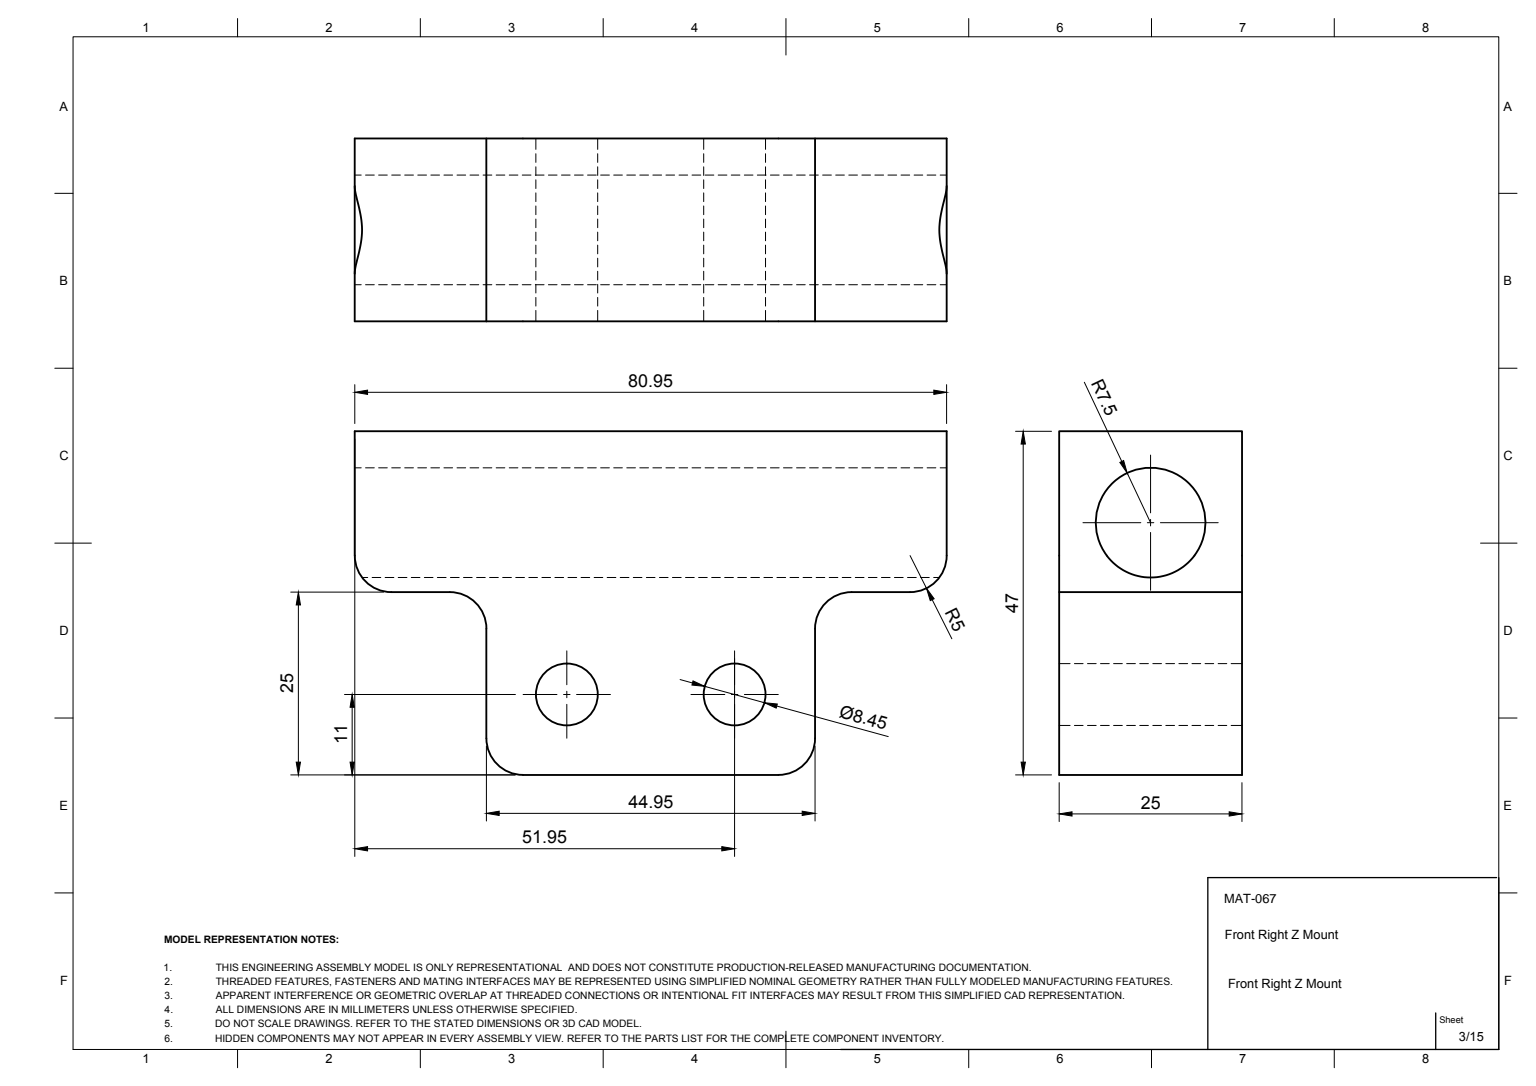
ISO-10303-21;
HEADER;
/* Generated by software containing ST-Developer
 * from STEP Tools, Inc. (www.steptools.com) 
 */

FILE_DESCRIPTION(
/* description */ ('CAx-IF Rec.Pracs.---Representation and Presentation of Product Manufa
cturing Information (PMI)---4.0---2014-10-13'),
/* implementation_level */ '2;1');

FILE_NAME(
/* name */ 'Front Right Z Mount.step',
/* time_stamp */ '2026-10-24T16:02:03-07:00',
/* author */ (''),
/* organization */ (''),
/* preprocessor_version */ 'ST-DEVELOPER v20.2',
/* originating_system */ 'Autodesk Translation Framework v15.17.0.0',
/* authorisation */ '');

FILE_SCHEMA (('AP242_MANAGED_MODEL_BASED_3D_ENGINEERING_MIM_LF { 1 0 10303 442 2 1 4 }'));
ENDSEC;

DATA;
#10=MECHANICAL_DESIGN_GEOMETRIC_PRESENTATION_REPRESENTATION('',(#349),#6348);
#327=SHAPE_REPRESENTATION_RELATIONSHIP('SRR','None',#6477,#338);
#338=ADVANCED_BREP_SHAPE_REPRESENTATION('',(#360),#6325);
#349=STYLED_ITEM('',(#6601),#360);
#360=MANIFOLD_SOLID_BREP('Body1',#3388);
#371=B_SPLINE_CURVE_WITH_KNOTS('',3,(#5227,#5228,#5229,#5230,#5231,#5232,
#5233,#5234,#5235,#5236,#5237,#5238,#5239,#5240,#5241,#5242,#5243,#5244),
 .UNSPECIFIED.,.F.,.F.,(4,2,2,2,2,2,2,2,4),(3.70111917994048,3.77979672158967,
4.08163951097076,4.2325609056613,4.38348230035184,4.53440369504239,4.68532508973293,
4.98716787911402,5.06584542076321),.UNSPECIFIED.);
#372=B_SPLINE_CURVE_WITH_KNOTS('',3,(#5245,#5246,#5247,#5248,#5249,#5250,
#5251,#5252,#5253,#5254,#5255,#5256,#5257,#5258,#5259,#5260,#5261,#5262),
 .UNSPECIFIED.,.F.,.F.,(4,2,2,2,2,2,2,2,4),(0.778797646372586,0.857475188021775,
1.15931797740286,1.31023937209341,1.46116076678395,1.61208216147449,1.76300355616504,
2.06484634554612,2.14352388719531),.UNSPECIFIED.);
#385=CYLINDRICAL_SURFACE('',#3548,0.004225);
#386=CYLINDRICAL_SURFACE('',#3549,0.004225);
#387=CYLINDRICAL_SURFACE('',#3551,0.0075);
#388=CYLINDRICAL_SURFACE('',#3556,0.005);
#389=CYLINDRICAL_SURFACE('',#3557,0.005);
#390=CYLINDRICAL_SURFACE('',#3558,0.005);
#391=CYLINDRICAL_SURFACE('',#3559,0.005);
#392=CYLINDRICAL_SURFACE('',#3560,0.005);
#393=CYLINDRICAL_SURFACE('',#3561,0.005);
#464=FACE_BOUND('',#869,.T.);
#465=FACE_BOUND('',#870,.T.);
#466=FACE_BOUND('',#872,.T.);
#467=FACE_BOUND('',#873,.T.);
#506=CIRCLE('',#3525,0.0075);
#507=CIRCLE('',#3526,0.0075);
#508=CIRCLE('',#3528,0.0075);
#509=CIRCLE('',#3529,0.0075);
#510=CIRCLE('',#3531,0.005);
#511=CIRCLE('',#3532,0.005);
#512=CIRCLE('',#3533,0.005);
#513=CIRCLE('',#3534,0.005);
#514=CIRCLE('',#3535,0.005);
#515=CIRCLE('',#3536,0.005);
#516=CIRCLE('',#3537,0.004225);
#517=CIRCLE('',#3538,0.004225);
#518=CIRCLE('',#3540,0.005);
#519=CIRCLE('',#3541,0.005);
#520=CIRCLE('',#3542,0.005);
#521=CIRCLE('',#3543,0.005);
#522=CIRCLE('',#3544,0.005);
#523=CIRCLE('',#3545,0.005);
#524=CIRCLE('',#3546,0.004225);
#525=CIRCLE('',#3547,0.004225);
#694=FACE_OUTER_BOUND('',#865,.T.);
#695=FACE_OUTER_BOUND('',#866,.T.);
#696=FACE_OUTER_BOUND('',#867,.T.);
#697=FACE_OUTER_BOUND('',#868,.T.);
#698=FACE_OUTER_BOUND('',#871,.T.);
#699=FACE_OUTER_BOUND('',#874,.T.);
#700=FACE_OUTER_BOUND('',#875,.T.);
#701=FACE_OUTER_BOUND('',#876,.T.);
#702=FACE_OUTER_BOUND('',#877,.T.);
#703=FACE_OUTER_BOUND('',#878,.T.);
#704=FACE_OUTER_BOUND('',#879,.T.);
#705=FACE_OUTER_BOUND('',#880,.T.);
#706=FACE_OUTER_BOUND('',#881,.T.);
#707=FACE_OUTER_BOUND('',#882,.T.);
#708=FACE_OUTER_BOUND('',#883,.T.);
#709=FACE_OUTER_BOUND('',#884,.T.);
#710=FACE_OUTER_BOUND('',#885,.T.);
#711=FACE_OUTER_BOUND('',#886,.T.);
#712=FACE_OUTER_BOUND('',#887,.T.);
#865=EDGE_LOOP('',(#2267,#2268,#2269,#2270));
#866=EDGE_LOOP('',(#2271,#2272,#2273,#2274,#2275,#2276,#2277));
#867=EDGE_LOOP('',(#2278,#2279,#2280,#2281,#2282,#2283,#2284));
#868=EDGE_LOOP('',(#2285,#2286,#2287,#2288,#2289,#2290,#2291,#2292,#2293,
#2294,#2295,#2296,#2297,#2298));
#869=EDGE_LOOP('',(#2299));
#870=EDGE_LOOP('',(#2300));
#871=EDGE_LOOP('',(#2301,#2302,#2303,#2304,#2305,#2306,#2307,#2308,#2309,
#2310,#2311,#2312,#2313,#2314));
#872=EDGE_LOOP('',(#2315));
#873=EDGE_LOOP('',(#2316));
#874=EDGE_LOOP('',(#2317,#2318,#2319,#2320));
#875=EDGE_LOOP('',(#2321,#2322,#2323,#2324));
#876=EDGE_LOOP('',(#2325,#2326,#2327,#2328));
#877=EDGE_LOOP('',(#2329,#2330,#2331,#2332,#2333,#2334,#2335,#2336));
#878=EDGE_LOOP('',(#2337,#2338,#2339,#2340));
#879=EDGE_LOOP('',(#2341,#2342,#2343,#2344));
#880=EDGE_LOOP('',(#2345,#2346,#2347,#2348));
#881=EDGE_LOOP('',(#2349,#2350,#2351,#2352));
#882=EDGE_LOOP('',(#2353,#2354,#2355,#2356));
#883=EDGE_LOOP('',(#2357,#2358,#2359,#2360,#2361,#2362));
#884=EDGE_LOOP('',(#2363,#2364,#2365,#2366));
#885=EDGE_LOOP('',(#2367,#2368,#2369,#2370,#2371,#2372));
#886=EDGE_LOOP('',(#2373,#2374,#2375,#2376));
#887=EDGE_LOOP('',(#2377,#2378,#2379,#2380));
#1078=LINE('',#5136,#1311);
#1079=LINE('',#5138,#1312);
#1080=LINE('',#5140,#1313);
#1081=LINE('',#5141,#1314);
#1082=LINE('',#5145,#1315);
#1083=LINE('',#5147,#1316);
#1084=LINE('',#5149,#1317);
#1085=LINE('',#5151,#1318);
#1086=LINE('',#5156,#1319);
#1087=LINE('',#5160,#1320);
#1088=LINE('',#5162,#1321);
#1089=LINE('',#5164,#1322);
#1090=LINE('',#5166,#1323);
#1091=LINE('',#5171,#1324);
#1092=LINE('',#5176,#1325);
#1093=LINE('',#5180,#1326);
#1094=LINE('',#5182,#1327);
#1095=LINE('',#5186,#1328);
#1096=LINE('',#5190,#1329);
#1097=LINE('',#5199,#1330);
#1098=LINE('',#5203,#1331);
#1099=LINE('',#5205,#1332);
#1100=LINE('',#5209,#1333);
#1101=LINE('',#5213,#1334);
#1102=LINE('',#5221,#1335);
#1103=LINE('',#5223,#1336);
#1104=LINE('',#5226,#1337);
#1105=LINE('',#5264,#1338);
#1106=LINE('',#5265,#1339);
#1107=LINE('',#5267,#1340);
#1108=LINE('',#5268,#1341);
#1109=LINE('',#5270,#1342);
#1110=LINE('',#5271,#1343);
#1111=LINE('',#5273,#1344);
#1112=LINE('',#5274,#1345);
#1311=VECTOR('',#3986,1.);
#1312=VECTOR('',#3987,1.);
#1313=VECTOR('',#3988,1.);
#1314=VECTOR('',#3989,1.);
#1315=VECTOR('',#3992,1.);
#1316=VECTOR('',#3993,1.);
#1317=VECTOR('',#3994,1.);
#1318=VECTOR('',#3995,1.);
#1319=VECTOR('',#4000,1.);
#1320=VECTOR('',#4003,1.);
#1321=VECTOR('',#4004,1.);
#1322=VECTOR('',#4005,1.);
#1323=VECTOR('',#4006,1.);
#1324=VECTOR('',#4011,1.);
#1325=VECTOR('',#4016,1.);
#1326=VECTOR('',#4019,1.);
#1327=VECTOR('',#4022,1.);
#1328=VECTOR('',#4025,1.);
#1329=VECTOR('',#4028,1.);
#1330=VECTOR('',#4037,1.);
#1331=VECTOR('',#4040,1.);
#1332=VECTOR('',#4043,1.);
#1333=VECTOR('',#4046,1.);
#1334=VECTOR('',#4049,1.);
#1335=VECTOR('',#4060,0.004225);
#1336=VECTOR('',#4063,0.004225);
#1337=VECTOR('',#4068,0.0075);
#1338=VECTOR('',#4071,1.);
#1339=VECTOR('',#4072,1.);
#1340=VECTOR('',#4075,1.);
#1341=VECTOR('',#4076,1.);
#1342=VECTOR('',#4079,1.);
#1343=VECTOR('',#4080,1.);
#1344=VECTOR('',#4083,1.);
#1345=VECTOR('',#4084,1.);
#1544=VERTEX_POINT('',#5134);
#1545=VERTEX_POINT('',#5135);
#1546=VERTEX_POINT('',#5137);
#1547=VERTEX_POINT('',#5139);
#1548=VERTEX_POINT('',#5143);
#1549=VERTEX_POINT('',#5144);
#1550=VERTEX_POINT('',#5146);
#1551=VERTEX_POINT('',#5148);
#1552=VERTEX_POINT('',#5150);
#1553=VERTEX_POINT('',#5152);
#1554=VERTEX_POINT('',#5154);
#1555=VERTEX_POINT('',#5158);
#1556=VERTEX_POINT('',#5159);
#1557=VERTEX_POINT('',#5161);
#1558=VERTEX_POINT('',#5163);
#1559=VERTEX_POINT('',#5165);
#1560=VERTEX_POINT('',#5167);
#1561=VERTEX_POINT('',#5169);
#1562=VERTEX_POINT('',#5173);
#1563=VERTEX_POINT('',#5175);
#1564=VERTEX_POINT('',#5177);
#1565=VERTEX_POINT('',#5179);
#1566=VERTEX_POINT('',#5183);
#1567=VERTEX_POINT('',#5185);
#1568=VERTEX_POINT('',#5187);
#1569=VERTEX_POINT('',#5189);
#1570=VERTEX_POINT('',#5192);
#1571=VERTEX_POINT('',#5194);
#1572=VERTEX_POINT('',#5197);
#1573=VERTEX_POINT('',#5198);
#1574=VERTEX_POINT('',#5200);
#1575=VERTEX_POINT('',#5202);
#1576=VERTEX_POINT('',#5206);
#1577=VERTEX_POINT('',#5208);
#1578=VERTEX_POINT('',#5210);
#1579=VERTEX_POINT('',#5212);
#1580=VERTEX_POINT('',#5216);
#1581=VERTEX_POINT('',#5218);
#1832=EDGE_CURVE('',#1544,#1545,#1078,.T.);
#1833=EDGE_CURVE('',#1546,#1544,#1079,.F.);
#1834=EDGE_CURVE('',#1546,#1547,#1080,.T.);
#1835=EDGE_CURVE('',#1545,#1547,#1081,.T.);
#1836=EDGE_CURVE('',#1548,#1549,#1082,.T.);
#1837=EDGE_CURVE('',#1549,#1550,#1083,.T.);
#1838=EDGE_CURVE('',#1551,#1550,#1084,.T.);
#1839=EDGE_CURVE('',#1552,#1551,#1085,.F.);
#1840=EDGE_CURVE('',#1553,#1552,#506,.T.);
#1841=EDGE_CURVE('',#1554,#1553,#507,.T.);
#1842=EDGE_CURVE('',#1548,#1554,#1086,.F.);
#1843=EDGE_CURVE('',#1555,#1556,#1087,.T.);
#1844=EDGE_CURVE('',#1557,#1556,#1088,.T.);
#1845=EDGE_CURVE('',#1558,#1557,#1089,.T.);
#1846=EDGE_CURVE('',#1559,#1558,#1090,.T.);
#1847=EDGE_CURVE('',#1559,#1560,#508,.T.);
#1848=EDGE_CURVE('',#1560,#1561,#509,.T.);
#1849=EDGE_CURVE('',#1555,#1561,#1091,.T.);
#1850=EDGE_CURVE('',#1562,#1546,#510,.T.);
#1851=EDGE_CURVE('',#1562,#1563,#1092,.T.);
#1852=EDGE_CURVE('',#1564,#1563,#511,.F.);
#1853=EDGE_CURVE('',#1565,#1564,#1093,.T.);
#1854=EDGE_CURVE('',#1558,#1565,#512,.T.);
#1855=EDGE_CURVE('',#1557,#1549,#1094,.T.);
#1856=EDGE_CURVE('',#1566,#1548,#513,.T.);
#1857=EDGE_CURVE('',#1566,#1567,#1095,.T.);
#1858=EDGE_CURVE('',#1568,#1567,#514,.F.);
#1859=EDGE_CURVE('',#1569,#1568,#1096,.T.);
#1860=EDGE_CURVE('',#1547,#1569,#515,.T.);
#1861=EDGE_CURVE('',#1570,#1570,#516,.T.);
#1862=EDGE_CURVE('',#1571,#1571,#517,.T.);
#1863=EDGE_CURVE('',#1572,#1573,#1097,.T.);
#1864=EDGE_CURVE('',#1574,#1573,#518,.T.);
#1865=EDGE_CURVE('',#1575,#1574,#1098,.T.);
#1866=EDGE_CURVE('',#1551,#1575,#519,.F.);
#1867=EDGE_CURVE('',#1556,#1550,#1099,.T.);
#1868=EDGE_CURVE('',#1576,#1555,#520,.F.);
#1869=EDGE_CURVE('',#1576,#1577,#1100,.T.);
#1870=EDGE_CURVE('',#1578,#1577,#521,.T.);
#1871=EDGE_CURVE('',#1579,#1578,#1101,.T.);
#1872=EDGE_CURVE('',#1544,#1579,#522,.F.);
#1873=EDGE_CURVE('',#1572,#1545,#523,.F.);
#1874=EDGE_CURVE('',#1580,#1580,#524,.T.);
#1875=EDGE_CURVE('',#1581,#1581,#525,.T.);
#1876=EDGE_CURVE('',#1570,#1580,#1102,.T.);
#1877=EDGE_CURVE('',#1571,#1581,#1103,.T.);
#1878=EDGE_CURVE('',#1553,#1560,#1104,.T.);
#1879=EDGE_CURVE('',#1561,#1559,#371,.T.);
#1880=EDGE_CURVE('',#1554,#1552,#372,.T.);
#1881=EDGE_CURVE('',#1573,#1568,#1105,.T.);
#1882=EDGE_CURVE('',#1569,#1572,#1106,.F.);
#1883=EDGE_CURVE('',#1567,#1574,#1107,.F.);
#1884=EDGE_CURVE('',#1575,#1566,#1108,.T.);
#1885=EDGE_CURVE('',#1579,#1562,#1109,.T.);
#1886=EDGE_CURVE('',#1563,#1578,#1110,.F.);
#1887=EDGE_CURVE('',#1577,#1564,#1111,.T.);
#1888=EDGE_CURVE('',#1565,#1576,#1112,.F.);
#2267=ORIENTED_EDGE('',*,*,#1832,.F.);
#2268=ORIENTED_EDGE('',*,*,#1833,.F.);
#2269=ORIENTED_EDGE('',*,*,#1834,.T.);
#2270=ORIENTED_EDGE('',*,*,#1835,.F.);
#2271=ORIENTED_EDGE('',*,*,#1836,.T.);
#2272=ORIENTED_EDGE('',*,*,#1837,.T.);
#2273=ORIENTED_EDGE('',*,*,#1838,.F.);
#2274=ORIENTED_EDGE('',*,*,#1839,.F.);
#2275=ORIENTED_EDGE('',*,*,#1840,.F.);
#2276=ORIENTED_EDGE('',*,*,#1841,.F.);
#2277=ORIENTED_EDGE('',*,*,#1842,.F.);
#2278=ORIENTED_EDGE('',*,*,#1843,.T.);
#2279=ORIENTED_EDGE('',*,*,#1844,.F.);
#2280=ORIENTED_EDGE('',*,*,#1845,.F.);
#2281=ORIENTED_EDGE('',*,*,#1846,.F.);
#2282=ORIENTED_EDGE('',*,*,#1847,.T.);
#2283=ORIENTED_EDGE('',*,*,#1848,.T.);
#2284=ORIENTED_EDGE('',*,*,#1849,.F.);
#2285=ORIENTED_EDGE('',*,*,#1834,.F.);
#2286=ORIENTED_EDGE('',*,*,#1850,.F.);
#2287=ORIENTED_EDGE('',*,*,#1851,.T.);
#2288=ORIENTED_EDGE('',*,*,#1852,.F.);
#2289=ORIENTED_EDGE('',*,*,#1853,.F.);
#2290=ORIENTED_EDGE('',*,*,#1854,.F.);
#2291=ORIENTED_EDGE('',*,*,#1845,.T.);
#2292=ORIENTED_EDGE('',*,*,#1855,.T.);
#2293=ORIENTED_EDGE('',*,*,#1836,.F.);
#2294=ORIENTED_EDGE('',*,*,#1856,.F.);
#2295=ORIENTED_EDGE('',*,*,#1857,.T.);
#2296=ORIENTED_EDGE('',*,*,#1858,.F.);
#2297=ORIENTED_EDGE('',*,*,#1859,.F.);
#2298=ORIENTED_EDGE('',*,*,#1860,.F.);
#2299=ORIENTED_EDGE('',*,*,#1861,.T.);
#2300=ORIENTED_EDGE('',*,*,#1862,.T.);
#2301=ORIENTED_EDGE('',*,*,#1863,.T.);
#2302=ORIENTED_EDGE('',*,*,#1864,.F.);
#2303=ORIENTED_EDGE('',*,*,#1865,.F.);
#2304=ORIENTED_EDGE('',*,*,#1866,.F.);
#2305=ORIENTED_EDGE('',*,*,#1838,.T.);
#2306=ORIENTED_EDGE('',*,*,#1867,.F.);
#2307=ORIENTED_EDGE('',*,*,#1843,.F.);
#2308=ORIENTED_EDGE('',*,*,#1868,.F.);
#2309=ORIENTED_EDGE('',*,*,#1869,.T.);
#2310=ORIENTED_EDGE('',*,*,#1870,.F.);
#2311=ORIENTED_EDGE('',*,*,#1871,.F.);
#2312=ORIENTED_EDGE('',*,*,#1872,.F.);
#2313=ORIENTED_EDGE('',*,*,#1832,.T.);
#2314=ORIENTED_EDGE('',*,*,#1873,.F.);
#2315=ORIENTED_EDGE('',*,*,#1874,.F.);
#2316=ORIENTED_EDGE('',*,*,#1875,.F.);
#2317=ORIENTED_EDGE('',*,*,#1861,.F.);
#2318=ORIENTED_EDGE('',*,*,#1876,.T.);
#2319=ORIENTED_EDGE('',*,*,#1874,.T.);
#2320=ORIENTED_EDGE('',*,*,#1876,.F.);
#2321=ORIENTED_EDGE('',*,*,#1862,.F.);
#2322=ORIENTED_EDGE('',*,*,#1877,.T.);
#2323=ORIENTED_EDGE('',*,*,#1875,.T.);
#2324=ORIENTED_EDGE('',*,*,#1877,.F.);
#2325=ORIENTED_EDGE('',*,*,#1867,.T.);
#2326=ORIENTED_EDGE('',*,*,#1837,.F.);
#2327=ORIENTED_EDGE('',*,*,#1855,.F.);
#2328=ORIENTED_EDGE('',*,*,#1844,.T.);
#2329=ORIENTED_EDGE('',*,*,#1841,.T.);
#2330=ORIENTED_EDGE('',*,*,#1878,.T.);
#2331=ORIENTED_EDGE('',*,*,#1847,.F.);
#2332=ORIENTED_EDGE('',*,*,#1879,.F.);
#2333=ORIENTED_EDGE('',*,*,#1848,.F.);
#2334=ORIENTED_EDGE('',*,*,#1878,.F.);
#2335=ORIENTED_EDGE('',*,*,#1840,.T.);
#2336=ORIENTED_EDGE('',*,*,#1880,.F.);
#2337=ORIENTED_EDGE('',*,*,#1859,.T.);
#2338=ORIENTED_EDGE('',*,*,#1881,.F.);
#2339=ORIENTED_EDGE('',*,*,#1863,.F.);
#2340=ORIENTED_EDGE('',*,*,#1882,.F.);
#2341=ORIENTED_EDGE('',*,*,#1865,.T.);
#2342=ORIENTED_EDGE('',*,*,#1883,.F.);
#2343=ORIENTED_EDGE('',*,*,#1857,.F.);
#2344=ORIENTED_EDGE('',*,*,#1884,.F.);
#2345=ORIENTED_EDGE('',*,*,#1851,.F.);
#2346=ORIENTED_EDGE('',*,*,#1885,.F.);
#2347=ORIENTED_EDGE('',*,*,#1871,.T.);
#2348=ORIENTED_EDGE('',*,*,#1886,.F.);
#2349=ORIENTED_EDGE('',*,*,#1853,.T.);
#2350=ORIENTED_EDGE('',*,*,#1887,.F.);
#2351=ORIENTED_EDGE('',*,*,#1869,.F.);
#2352=ORIENTED_EDGE('',*,*,#1888,.F.);
#2353=ORIENTED_EDGE('',*,*,#1873,.T.);
#2354=ORIENTED_EDGE('',*,*,#1835,.T.);
#2355=ORIENTED_EDGE('',*,*,#1860,.T.);
#2356=ORIENTED_EDGE('',*,*,#1882,.T.);
#2357=ORIENTED_EDGE('',*,*,#1880,.T.);
#2358=ORIENTED_EDGE('',*,*,#1839,.T.);
#2359=ORIENTED_EDGE('',*,*,#1866,.T.);
#2360=ORIENTED_EDGE('',*,*,#1884,.T.);
#2361=ORIENTED_EDGE('',*,*,#1856,.T.);
#2362=ORIENTED_EDGE('',*,*,#1842,.T.);
#2363=ORIENTED_EDGE('',*,*,#1864,.T.);
#2364=ORIENTED_EDGE('',*,*,#1881,.T.);
#2365=ORIENTED_EDGE('',*,*,#1858,.T.);
#2366=ORIENTED_EDGE('',*,*,#1883,.T.);
#2367=ORIENTED_EDGE('',*,*,#1868,.T.);
#2368=ORIENTED_EDGE('',*,*,#1849,.T.);
#2369=ORIENTED_EDGE('',*,*,#1879,.T.);
#2370=ORIENTED_EDGE('',*,*,#1846,.T.);
#2371=ORIENTED_EDGE('',*,*,#1854,.T.);
#2372=ORIENTED_EDGE('',*,*,#1888,.T.);
#2373=ORIENTED_EDGE('',*,*,#1870,.T.);
#2374=ORIENTED_EDGE('',*,*,#1887,.T.);
#2375=ORIENTED_EDGE('',*,*,#1852,.T.);
#2376=ORIENTED_EDGE('',*,*,#1886,.T.);
#2377=ORIENTED_EDGE('',*,*,#1872,.T.);
#2378=ORIENTED_EDGE('',*,*,#1885,.T.);
#2379=ORIENTED_EDGE('',*,*,#1850,.T.);
#2380=ORIENTED_EDGE('',*,*,#1833,.T.);
#3137=PLANE('',#3523);
#3138=PLANE('',#3524);
#3139=PLANE('',#3527);
#3140=PLANE('',#3530);
#3141=PLANE('',#3539);
#3142=PLANE('',#3550);
#3143=PLANE('',#3552);
#3144=PLANE('',#3553);
#3145=PLANE('',#3554);
#3146=PLANE('',#3555);
#3217=ADVANCED_FACE('',(#694),#3137,.F.);
#3218=ADVANCED_FACE('',(#695),#3138,.F.);
#3219=ADVANCED_FACE('',(#696),#3139,.T.);
#3220=ADVANCED_FACE('',(#697,#464,#465),#3140,.T.);
#3221=ADVANCED_FACE('',(#698,#466,#467),#3141,.F.);
#3222=ADVANCED_FACE('',(#699),#385,.F.);
#3223=ADVANCED_FACE('',(#700),#386,.F.);
#3224=ADVANCED_FACE('',(#701),#3142,.T.);
#3225=ADVANCED_FACE('',(#702),#387,.F.);
#3226=ADVANCED_FACE('',(#703),#3143,.T.);
#3227=ADVANCED_FACE('',(#704),#3144,.F.);
#3228=ADVANCED_FACE('',(#705),#3145,.F.);
#3229=ADVANCED_FACE('',(#706),#3146,.T.);
#3230=ADVANCED_FACE('',(#707),#388,.T.);
#3231=ADVANCED_FACE('',(#708),#389,.T.);
#3232=ADVANCED_FACE('',(#709),#390,.F.);
#3233=ADVANCED_FACE('',(#710),#391,.T.);
#3234=ADVANCED_FACE('',(#711),#392,.F.);
#3235=ADVANCED_FACE('',(#712),#393,.T.);
#3388=CLOSED_SHELL('',(#3217,#3218,#3219,#3220,#3221,#3222,#3223,#3224,
#3225,#3226,#3227,#3228,#3229,#3230,#3231,#3232,#3233,#3234,#3235));
#3522=AXIS2_PLACEMENT_3D('',#5132,#3982,#3983);
#3523=AXIS2_PLACEMENT_3D('',#5133,#3984,#3985);
#3524=AXIS2_PLACEMENT_3D('',#5142,#3990,#3991);
#3525=AXIS2_PLACEMENT_3D('',#5153,#3996,#3997);
#3526=AXIS2_PLACEMENT_3D('',#5155,#3998,#3999);
#3527=AXIS2_PLACEMENT_3D('',#5157,#4001,#4002);
#3528=AXIS2_PLACEMENT_3D('',#5168,#4007,#4008);
#3529=AXIS2_PLACEMENT_3D('',#5170,#4009,#4010);
#3530=AXIS2_PLACEMENT_3D('',#5172,#4012,#4013);
#3531=AXIS2_PLACEMENT_3D('',#5174,#4014,#4015);
#3532=AXIS2_PLACEMENT_3D('',#5178,#4017,#4018);
#3533=AXIS2_PLACEMENT_3D('',#5181,#4020,#4021);
#3534=AXIS2_PLACEMENT_3D('',#5184,#4023,#4024);
#3535=AXIS2_PLACEMENT_3D('',#5188,#4026,#4027);
#3536=AXIS2_PLACEMENT_3D('',#5191,#4029,#4030);
#3537=AXIS2_PLACEMENT_3D('',#5193,#4031,#4032);
#3538=AXIS2_PLACEMENT_3D('',#5195,#4033,#4034);
#3539=AXIS2_PLACEMENT_3D('',#5196,#4035,#4036);
#3540=AXIS2_PLACEMENT_3D('',#5201,#4038,#4039);
#3541=AXIS2_PLACEMENT_3D('',#5204,#4041,#4042);
#3542=AXIS2_PLACEMENT_3D('',#5207,#4044,#4045);
#3543=AXIS2_PLACEMENT_3D('',#5211,#4047,#4048);
#3544=AXIS2_PLACEMENT_3D('',#5214,#4050,#4051);
#3545=AXIS2_PLACEMENT_3D('',#5215,#4052,#4053);
#3546=AXIS2_PLACEMENT_3D('',#5217,#4054,#4055);
#3547=AXIS2_PLACEMENT_3D('',#5219,#4056,#4057);
#3548=AXIS2_PLACEMENT_3D('',#5220,#4058,#4059);
#3549=AXIS2_PLACEMENT_3D('',#5222,#4061,#4062);
#3550=AXIS2_PLACEMENT_3D('',#5224,#4064,#4065);
#3551=AXIS2_PLACEMENT_3D('',#5225,#4066,#4067);
#3552=AXIS2_PLACEMENT_3D('',#5263,#4069,#4070);
#3553=AXIS2_PLACEMENT_3D('',#5266,#4073,#4074);
#3554=AXIS2_PLACEMENT_3D('',#5269,#4077,#4078);
#3555=AXIS2_PLACEMENT_3D('',#5272,#4081,#4082);
#3556=AXIS2_PLACEMENT_3D('',#5275,#4085,#4086);
#3557=AXIS2_PLACEMENT_3D('',#5276,#4087,#4088);
#3558=AXIS2_PLACEMENT_3D('',#5277,#4089,#4090);
#3559=AXIS2_PLACEMENT_3D('',#5278,#4091,#4092);
#3560=AXIS2_PLACEMENT_3D('',#5279,#4093,#4094);
#3561=AXIS2_PLACEMENT_3D('',#5280,#4095,#4096);
#3982=DIRECTION('axis',(0.,0.,1.));
#3983=DIRECTION('refdir',(1.,0.,0.));
#3984=DIRECTION('center_axis',(-1.,0.,0.));
#3985=DIRECTION('ref_axis',(0.,0.,-1.));
#3986=DIRECTION('',(0.,-8.57182693503055E-17,-1.));
#3987=DIRECTION('',(0.,-1.,8.57182693503055E-17));
#3988=DIRECTION('',(0.,-8.57182693503055E-17,-1.));
#3989=DIRECTION('',(0.,-1.,8.57182693503055E-17));
#3990=DIRECTION('center_axis',(0.,8.57182693503055E-17,1.));
#3991=DIRECTION('ref_axis',(0.,-1.,8.57182693503055E-17));
#3992=DIRECTION('',(-1.,0.,0.));
#3993=DIRECTION('',(0.,1.,-8.57182693503055E-17));
#3994=DIRECTION('',(-1.,0.,0.));
#3995=DIRECTION('',(0.,-1.,8.57182693503055E-17));
#3996=DIRECTION('center_axis',(0.,-8.57182693503055E-17,-1.));
#3997=DIRECTION('ref_axis',(0.,-1.,8.57182693503055E-17));
#3998=DIRECTION('center_axis',(0.,-8.57182693503055E-17,-1.));
#3999=DIRECTION('ref_axis',(0.,-1.,8.57182693503055E-17));
#4000=DIRECTION('',(0.,-1.,8.57182693503055E-17));
#4001=DIRECTION('center_axis',(0.,8.57182693503055E-17,1.));
#4002=DIRECTION('ref_axis',(0.,-1.,8.57182693503055E-17));
#4003=DIRECTION('',(-1.,0.,0.));
#4004=DIRECTION('',(0.,1.,-8.57182693503055E-17));
#4005=DIRECTION('',(-1.,0.,0.));
#4006=DIRECTION('',(0.,-1.,8.57182693503055E-17));
#4007=DIRECTION('center_axis',(0.,-8.57182693503055E-17,-1.));
#4008=DIRECTION('ref_axis',(0.,-1.,8.57182693503055E-17));
#4009=DIRECTION('center_axis',(0.,-8.57182693503055E-17,-1.));
#4010=DIRECTION('ref_axis',(0.,-1.,8.57182693503055E-17));
#4011=DIRECTION('',(0.,-1.,8.57182693503055E-17));
#4012=DIRECTION('center_axis',(0.,-1.,8.57182693503055E-17));
#4013=DIRECTION('ref_axis',(-1.,0.,0.));
#4014=DIRECTION('center_axis',(0.,1.,-8.57182693503055E-17));
#4015=DIRECTION('ref_axis',(0.,-8.57182693503055E-17,-1.));
#4016=DIRECTION('',(-1.,0.,0.));
#4017=DIRECTION('center_axis',(0.,1.,-8.57182693503055E-17));
#4018=DIRECTION('ref_axis',(0.,-8.57182693503055E-17,-1.));
#4019=DIRECTION('',(0.,-8.57182693503055E-17,-1.));
#4020=DIRECTION('center_axis',(0.,1.,-8.57182693503055E-17));
#4021=DIRECTION('ref_axis',(0.,-8.57182693503055E-17,-1.));
#4022=DIRECTION('',(0.,-8.57182693503055E-17,-1.));
#4023=DIRECTION('center_axis',(0.,1.,-8.57182693503055E-17));
#4024=DIRECTION('ref_axis',(0.,-8.57182693503055E-17,-1.));
#4025=DIRECTION('',(0.,8.57182693503055E-17,1.));
#4026=DIRECTION('center_axis',(0.,1.,-8.57182693503055E-17));
#4027=DIRECTION('ref_axis',(0.,-8.57182693503055E-17,-1.));
#4028=DIRECTION('',(-1.,0.,0.));
#4029=DIRECTION('center_axis',(0.,1.,-8.57182693503055E-17));
#4030=DIRECTION('ref_axis',(0.,-8.57182693503055E-17,-1.));
#4031=DIRECTION('center_axis',(0.,1.,-8.57182693503055E-17));
#4032=DIRECTION('ref_axis',(0.,-8.57182693503055E-17,-1.));
#4033=DIRECTION('center_axis',(0.,1.,-8.57182693503055E-17));
#4034=DIRECTION('ref_axis',(0.,-8.57182693503055E-17,-1.));
#4035=DIRECTION('center_axis',(0.,-1.,8.57182693503055E-17));
#4036=DIRECTION('ref_axis',(-1.,0.,0.));
#4037=DIRECTION('',(-1.,0.,0.));
#4038=DIRECTION('center_axis',(0.,1.,-8.57182693503055E-17));
#4039=DIRECTION('ref_axis',(0.,-8.57182693503055E-17,-1.));
#4040=DIRECTION('',(0.,8.57182693503055E-17,1.));
#4041=DIRECTION('center_axis',(0.,1.,-8.57182693503055E-17));
#4042=DIRECTION('ref_axis',(0.,-8.57182693503055E-17,-1.));
#4043=DIRECTION('',(0.,-8.57182693503055E-17,-1.));
#4044=DIRECTION('center_axis',(0.,1.,-8.57182693503055E-17));
#4045=DIRECTION('ref_axis',(0.,-8.57182693503055E-17,-1.));
#4046=DIRECTION('',(0.,-8.57182693503055E-17,-1.));
#4047=DIRECTION('center_axis',(0.,1.,-8.57182693503055E-17));
#4048=DIRECTION('ref_axis',(0.,-8.57182693503055E-17,-1.));
#4049=DIRECTION('',(-1.,0.,0.));
#4050=DIRECTION('center_axis',(0.,1.,-8.57182693503055E-17));
#4051=DIRECTION('ref_axis',(0.,-8.57182693503055E-17,-1.));
#4052=DIRECTION('center_axis',(0.,1.,-8.57182693503055E-17));
#4053=DIRECTION('ref_axis',(0.,-8.57182693503055E-17,-1.));
#4054=DIRECTION('center_axis',(0.,1.,-8.57182693503055E-17));
#4055=DIRECTION('ref_axis',(0.,-8.57182693503055E-17,-1.));
#4056=DIRECTION('center_axis',(0.,1.,-8.57182693503055E-17));
#4057=DIRECTION('ref_axis',(0.,-8.57182693503055E-17,-1.));
#4058=DIRECTION('center_axis',(0.,1.,-8.57182693503055E-17));
#4059=DIRECTION('ref_axis',(0.,8.57182693503055E-17,1.));
#4060=DIRECTION('',(0.,1.,-8.57182693503055E-17));
#4061=DIRECTION('center_axis',(0.,1.,-8.57182693503055E-17));
#4062=DIRECTION('ref_axis',(0.,8.57182693503055E-17,1.));
#4063=DIRECTION('',(0.,1.,-8.57182693503055E-17));
#4064=DIRECTION('center_axis',(-1.,0.,0.));
#4065=DIRECTION('ref_axis',(0.,0.,-1.));
#4066=DIRECTION('center_axis',(0.,8.57182693503055E-17,1.));
#4067=DIRECTION('ref_axis',(0.,-1.,8.57182693503055E-17));
#4068=DIRECTION('',(0.,8.57182693503055E-17,1.));
#4069=DIRECTION('center_axis',(0.,-8.57182693503055E-17,-1.));
#4070=DIRECTION('ref_axis',(0.,1.,-8.57182693503055E-17));
#4071=DIRECTION('',(0.,-1.,8.57182693503055E-17));
#4072=DIRECTION('',(0.,-1.,8.57182693503055E-17));
#4073=DIRECTION('center_axis',(-1.,0.,0.));
#4074=DIRECTION('ref_axis',(0.,0.,-1.));
#4075=DIRECTION('',(0.,-1.,8.57182693503055E-17));
#4076=DIRECTION('',(0.,-1.,8.57182693503055E-17));
#4077=DIRECTION('center_axis',(0.,-8.57182693503055E-17,-1.));
#4078=DIRECTION('ref_axis',(0.,1.,-8.57182693503055E-17));
#4079=DIRECTION('',(0.,-1.,8.57182693503055E-17));
#4080=DIRECTION('',(0.,-1.,8.57182693503055E-17));
#4081=DIRECTION('center_axis',(1.,0.,0.));
#4082=DIRECTION('ref_axis',(0.,0.,1.));
#4083=DIRECTION('',(0.,-1.,8.57182693503055E-17));
#4084=DIRECTION('',(0.,-1.,8.57182693503055E-17));
#4085=DIRECTION('center_axis',(0.,1.,-8.57182693503055E-17));
#4086=DIRECTION('ref_axis',(0.,8.57182693503055E-17,1.));
#4087=DIRECTION('center_axis',(0.,-1.,8.57182693503055E-17));
#4088=DIRECTION('ref_axis',(0.,-8.57182693503055E-17,-1.));
#4089=DIRECTION('center_axis',(0.,-1.,8.57182693503055E-17));
#4090=DIRECTION('ref_axis',(0.,-8.57182693503055E-17,-1.));
#4091=DIRECTION('center_axis',(0.,-1.,8.57182693503055E-17));
#4092=DIRECTION('ref_axis',(0.,-8.57182693503055E-17,-1.));
#4093=DIRECTION('center_axis',(0.,-1.,8.57182693503055E-17));
#4094=DIRECTION('ref_axis',(0.,-8.57182693503055E-17,-1.));
#4095=DIRECTION('center_axis',(0.,-1.,8.57182693503055E-17));
#4096=DIRECTION('ref_axis',(0.,-8.57182693503055E-17,-1.));
#5132=CARTESIAN_POINT('',(0.,0.,0.));
#5133=CARTESIAN_POINT('Origin',(0.06855,-0.1092,0.02565));
#5134=CARTESIAN_POINT('',(0.06855,-0.0842,0.043125));
#5135=CARTESIAN_POINT('',(0.06855,-0.0842,0.008175));
#5136=CARTESIAN_POINT('',(0.06855,-0.0842,0.02565));
#5137=CARTESIAN_POINT('',(0.06855,-0.1092,0.043125));
#5138=CARTESIAN_POINT('',(0.06855,-0.1092,0.043125));
#5139=CARTESIAN_POINT('',(0.06855,-0.1092,0.008175));
#5140=CARTESIAN_POINT('',(0.06855,-0.1092,0.02565));
#5141=CARTESIAN_POINT('',(0.06855,-0.1092,0.008175));
#5142=CARTESIAN_POINT('Origin',(0.05755,-0.1092,-0.014825));
#5143=CARTESIAN_POINT('',(0.03855,-0.1092,-0.014825));
#5144=CARTESIAN_POINT('',(0.02155,-0.1092,-0.014825));
#5145=CARTESIAN_POINT('',(0.05755,-0.1092,-0.014825));
#5146=CARTESIAN_POINT('',(0.02155,-0.0842,-0.014825));
#5147=CARTESIAN_POINT('',(0.02155,-0.1092,-0.014825));
#5148=CARTESIAN_POINT('',(0.03855,-0.0842,-0.014825));
#5149=CARTESIAN_POINT('',(0.05755,-0.0842,-0.014825));
#5150=CARTESIAN_POINT('',(0.03855,-0.0907,-0.014825));
#5151=CARTESIAN_POINT('',(0.03855,-0.1092,-0.014825));
#5152=CARTESIAN_POINT('',(0.03405,-0.0892,-0.014825));
#5153=CARTESIAN_POINT('Origin',(0.03405,-0.0967,-0.014825));
#5154=CARTESIAN_POINT('',(0.03855,-0.1027,-0.014825));
#5155=CARTESIAN_POINT('Origin',(0.03405,-0.0967,-0.014825));
#5156=CARTESIAN_POINT('',(0.03855,-0.1092,-0.014825));
#5157=CARTESIAN_POINT('Origin',(0.05755,-0.1092,0.066125));
#5158=CARTESIAN_POINT('',(0.03855,-0.0842,0.066125));
#5159=CARTESIAN_POINT('',(0.02155,-0.0842,0.066125));
#5160=CARTESIAN_POINT('',(0.05755,-0.0842,0.066125));
#5161=CARTESIAN_POINT('',(0.02155,-0.1092,0.066125));
#5162=CARTESIAN_POINT('',(0.02155,-0.1092,0.066125));
#5163=CARTESIAN_POINT('',(0.03855,-0.1092,0.066125));
#5164=CARTESIAN_POINT('',(0.05755,-0.1092,0.066125));
#5165=CARTESIAN_POINT('',(0.03855,-0.1027,0.066125));
#5166=CARTESIAN_POINT('',(0.03855,-0.1092,0.066125));
#5167=CARTESIAN_POINT('',(0.03405,-0.0892,0.066125));
#5168=CARTESIAN_POINT('Origin',(0.03405,-0.0967,0.066125));
#5169=CARTESIAN_POINT('',(0.03855,-0.0907,0.066125));
#5170=CARTESIAN_POINT('Origin',(0.03405,-0.0967,0.066125));
#5171=CARTESIAN_POINT('',(0.03855,-0.1092,0.066125));
#5172=CARTESIAN_POINT('Origin',(0.05755,-0.1092,0.02565));
#5173=CARTESIAN_POINT('',(0.06355,-0.1092,0.048125));
#5174=CARTESIAN_POINT('Origin',(0.06355,-0.1092,0.043125));
#5175=CARTESIAN_POINT('',(0.04855,-0.1092,0.048125));
#5176=CARTESIAN_POINT('',(0.05605,-0.1092,0.048125));
#5177=CARTESIAN_POINT('',(0.04355,-0.1092,0.053125));
#5178=CARTESIAN_POINT('Origin',(0.04855,-0.1092,0.053125));
#5179=CARTESIAN_POINT('',(0.04355,-0.1092,0.061125));
#5180=CARTESIAN_POINT('',(0.04355,-0.1092,0.057125));
#5181=CARTESIAN_POINT('Origin',(0.03855,-0.1092,0.061125));
#5182=CARTESIAN_POINT('',(0.02155,-0.1092,0.02565));
#5183=CARTESIAN_POINT('',(0.04355,-0.1092,-0.009825));
#5184=CARTESIAN_POINT('Origin',(0.03855,-0.1092,-0.009825));
#5185=CARTESIAN_POINT('',(0.04355,-0.1092,-0.001825));
#5186=CARTESIAN_POINT('',(0.04355,-0.1092,-0.005825));
#5187=CARTESIAN_POINT('',(0.04855,-0.1092,0.003175));
#5188=CARTESIAN_POINT('Origin',(0.04855,-0.1092,-0.001825));
#5189=CARTESIAN_POINT('',(0.06355,-0.1092,0.003175));
#5190=CARTESIAN_POINT('',(0.05605,-0.1092,0.003175));
#5191=CARTESIAN_POINT('Origin',(0.06355,-0.1092,0.008175));
#5192=CARTESIAN_POINT('',(0.05755,-0.1092,0.0329));
#5193=CARTESIAN_POINT('Origin',(0.05755,-0.1092,0.037125));
#5194=CARTESIAN_POINT('',(0.05755,-0.1092,0.00995));
#5195=CARTESIAN_POINT('Origin',(0.05755,-0.1092,0.014175));
#5196=CARTESIAN_POINT('Origin',(0.05755,-0.0842,0.02565));
#5197=CARTESIAN_POINT('',(0.06355,-0.0842,0.003175));
#5198=CARTESIAN_POINT('',(0.04855,-0.0842,0.003175));
#5199=CARTESIAN_POINT('',(0.05605,-0.0842,0.003175));
#5200=CARTESIAN_POINT('',(0.04355,-0.0842,-0.001825));
#5201=CARTESIAN_POINT('Origin',(0.04855,-0.0842,-0.001825));
#5202=CARTESIAN_POINT('',(0.04355,-0.0842,-0.009825));
#5203=CARTESIAN_POINT('',(0.04355,-0.0842,-0.005825));
#5204=CARTESIAN_POINT('Origin',(0.03855,-0.0842,-0.009825));
#5205=CARTESIAN_POINT('',(0.02155,-0.0842,0.02565));
#5206=CARTESIAN_POINT('',(0.04355,-0.0842,0.061125));
#5207=CARTESIAN_POINT('Origin',(0.03855,-0.0842,0.061125));
#5208=CARTESIAN_POINT('',(0.04355,-0.0842,0.053125));
#5209=CARTESIAN_POINT('',(0.04355,-0.0842,0.057125));
#5210=CARTESIAN_POINT('',(0.04855,-0.0842,0.048125));
#5211=CARTESIAN_POINT('Origin',(0.04855,-0.0842,0.053125));
#5212=CARTESIAN_POINT('',(0.06355,-0.0842,0.048125));
#5213=CARTESIAN_POINT('',(0.05605,-0.0842,0.048125));
#5214=CARTESIAN_POINT('Origin',(0.06355,-0.0842,0.043125));
#5215=CARTESIAN_POINT('Origin',(0.06355,-0.0842,0.008175));
#5216=CARTESIAN_POINT('',(0.05755,-0.0842,0.0329));
#5217=CARTESIAN_POINT('Origin',(0.05755,-0.0842,0.037125));
#5218=CARTESIAN_POINT('',(0.05755,-0.0842,0.00995));
#5219=CARTESIAN_POINT('Origin',(0.05755,-0.0842,0.014175));
#5220=CARTESIAN_POINT('Origin',(0.05755,-0.1092,0.037125));
#5221=CARTESIAN_POINT('',(0.05755,-0.1092,0.0329));
#5222=CARTESIAN_POINT('Origin',(0.05755,-0.1092,0.014175));
#5223=CARTESIAN_POINT('',(0.05755,-0.1092,0.00995));
#5224=CARTESIAN_POINT('Origin',(0.02155,-0.1092,0.02565));
#5225=CARTESIAN_POINT('Origin',(0.03405,-0.0967,-0.023875));
#5226=CARTESIAN_POINT('',(0.03405,-0.0892,-0.023875));
#5227=CARTESIAN_POINT('Ctrl Pts',(0.03855,-0.0907,0.066125));
#5228=CARTESIAN_POINT('Ctrl Pts',(0.0387729524989471,-0.0908672143742104,
0.066125));
#5229=CARTESIAN_POINT('Ctrl Pts',(0.0389827504953742,-0.0910443676288105,
0.0661099450879691));
#5230=CARTESIAN_POINT('Ctrl Pts',(0.0399051826894431,-0.0919072239369945,
0.0659940175331532));
#5231=CARTESIAN_POINT('Ctrl Pts',(0.0405168708018142,-0.0927639295079321,
0.0657455865368071));
#5232=CARTESIAN_POINT('Ctrl Pts',(0.0411335425015076,-0.0941822279651364,
0.0654121811456859));
#5233=CARTESIAN_POINT('Ctrl Pts',(0.0412904479475092,-0.0946775248634452,
0.0653090151899698));
#5234=CARTESIAN_POINT('Ctrl Pts',(0.0414987473161672,-0.0956847881043564,
0.065164916792468));
#5235=CARTESIAN_POINT('Ctrl Pts',(0.04155,-0.0961969286843649,0.065125));
#5236=CARTESIAN_POINT('Ctrl Pts',(0.04155,-0.0972030713156352,0.065125));
#5237=CARTESIAN_POINT('Ctrl Pts',(0.0414987473161672,-0.0977152118956436,
0.065164916792468));
#5238=CARTESIAN_POINT('Ctrl Pts',(0.0412904479475092,-0.0987224751365548,
0.0653090151899698));
#5239=CARTESIAN_POINT('Ctrl Pts',(0.0411335425015076,-0.0992177720348636,
0.0654121811456859));
#5240=CARTESIAN_POINT('Ctrl Pts',(0.0405168708018142,-0.100636070492068,
0.0657455865368071));
#5241=CARTESIAN_POINT('Ctrl Pts',(0.039905182689443,-0.101492776063005,
0.0659940175331532));
#5242=CARTESIAN_POINT('Ctrl Pts',(0.0389827504953742,-0.102355632371189,
0.0661099450879691));
#5243=CARTESIAN_POINT('Ctrl Pts',(0.0387729524989471,-0.10253278562579,
0.066125));
#5244=CARTESIAN_POINT('Ctrl Pts',(0.03855,-0.1027,0.066125));
#5245=CARTESIAN_POINT('Ctrl Pts',(0.03855,-0.1027,-0.014825));
#5246=CARTESIAN_POINT('Ctrl Pts',(0.0387729524989471,-0.10253278562579,
-0.014825));
#5247=CARTESIAN_POINT('Ctrl Pts',(0.0389827504953742,-0.102355632371189,
-0.0148099450879691));
#5248=CARTESIAN_POINT('Ctrl Pts',(0.0399051826894431,-0.101492776063005,
-0.0146940175331532));
#5249=CARTESIAN_POINT('Ctrl Pts',(0.0405168708018142,-0.100636070492068,
-0.0144455865368071));
#5250=CARTESIAN_POINT('Ctrl Pts',(0.0411335425015076,-0.0992177720348636,
-0.0141121811456859));
#5251=CARTESIAN_POINT('Ctrl Pts',(0.0412904479475092,-0.0987224751365548,
-0.0140090151899698));
#5252=CARTESIAN_POINT('Ctrl Pts',(0.0414987473161672,-0.0977152118956436,
-0.013864916792468));
#5253=CARTESIAN_POINT('Ctrl Pts',(0.04155,-0.0972030713156352,-0.013825));
#5254=CARTESIAN_POINT('Ctrl Pts',(0.04155,-0.0961969286843649,-0.013825));
#5255=CARTESIAN_POINT('Ctrl Pts',(0.0414987473161672,-0.0956847881043564,
-0.013864916792468));
#5256=CARTESIAN_POINT('Ctrl Pts',(0.0412904479475093,-0.0946775248634452,
-0.0140090151899698));
#5257=CARTESIAN_POINT('Ctrl Pts',(0.0411335425015076,-0.0941822279651364,
-0.0141121811456859));
#5258=CARTESIAN_POINT('Ctrl Pts',(0.0405168708018142,-0.0927639295079321,
-0.0144455865368071));
#5259=CARTESIAN_POINT('Ctrl Pts',(0.0399051826894431,-0.0919072239369945,
-0.0146940175331532));
#5260=CARTESIAN_POINT('Ctrl Pts',(0.0389827504953742,-0.0910443676288105,
-0.0148099450879691));
#5261=CARTESIAN_POINT('Ctrl Pts',(0.0387729524989471,-0.0908672143742103,
-0.014825));
#5262=CARTESIAN_POINT('Ctrl Pts',(0.03855,-0.0907,-0.014825));
#5263=CARTESIAN_POINT('Origin',(0.05605,-0.0842,0.003175));
#5264=CARTESIAN_POINT('',(0.04855,-0.0842,0.003175));
#5265=CARTESIAN_POINT('',(0.06355,-0.0842,0.003175));
#5266=CARTESIAN_POINT('Origin',(0.04355,-0.0842,-0.005825));
#5267=CARTESIAN_POINT('',(0.04355,-0.0842,-0.001825));
#5268=CARTESIAN_POINT('',(0.04355,-0.0842,-0.009825));
#5269=CARTESIAN_POINT('Origin',(0.05605,-0.0842,0.048125));
#5270=CARTESIAN_POINT('',(0.06355,-0.0842,0.048125));
#5271=CARTESIAN_POINT('',(0.04855,-0.0842,0.048125));
#5272=CARTESIAN_POINT('Origin',(0.04355,-0.0842,0.057125));
#5273=CARTESIAN_POINT('',(0.04355,-0.0842,0.053125));
#5274=CARTESIAN_POINT('',(0.04355,-0.0842,0.061125));
#5275=CARTESIAN_POINT('Origin',(0.06355,-0.1092,0.008175));
#5276=CARTESIAN_POINT('Origin',(0.03855,-0.0842,-0.009825));
#5277=CARTESIAN_POINT('Origin',(0.04855,-0.0842,-0.001825));
#5278=CARTESIAN_POINT('Origin',(0.03855,-0.1092,0.061125));
#5279=CARTESIAN_POINT('Origin',(0.04855,-0.0842,0.053125));
#5280=CARTESIAN_POINT('Origin',(0.06355,-0.0842,0.043125));
#6300=UNCERTAINTY_MEASURE_WITH_UNIT(LENGTH_MEASURE(1.E-5),#6349,
'DISTANCE_ACCURACY_VALUE',
'Maximum model space distance between geometric entities at asserted c
onnectivities');
#6323=UNCERTAINTY_MEASURE_WITH_UNIT(LENGTH_MEASURE(1.E-5),#6349,
'DISTANCE_ACCURACY_VALUE',
'Maximum model space distance between geometric entities at asserted c
onnectivities');
#6325=(
GEOMETRIC_REPRESENTATION_CONTEXT(3)
GLOBAL_UNCERTAINTY_ASSIGNED_CONTEXT((#6300))
GLOBAL_UNIT_ASSIGNED_CONTEXT((#6349,#6350,#6351))
REPRESENTATION_CONTEXT('','3D')
);
#6348=(
GEOMETRIC_REPRESENTATION_CONTEXT(3)
GLOBAL_UNCERTAINTY_ASSIGNED_CONTEXT((#6323))
GLOBAL_UNIT_ASSIGNED_CONTEXT((#6349,#6350,#6351))
REPRESENTATION_CONTEXT('','3D')
);
#6349=(
LENGTH_UNIT()
NAMED_UNIT(*)
SI_UNIT($,.METRE.)
);
#6350=(
NAMED_UNIT(*)
PLANE_ANGLE_UNIT()
SI_UNIT($,.RADIAN.)
);
#6351=(
NAMED_UNIT(*)
SI_UNIT($,.STERADIAN.)
SOLID_ANGLE_UNIT()
);
#6353=SHAPE_DEFINITION_REPRESENTATION(#6377,#6477);
#6377=PRODUCT_DEFINITION_SHAPE('',$,#6502);
#6477=SHAPE_REPRESENTATION('',(#3522),#6325);
#6500=PRODUCT_DEFINITION_CONTEXT('part definition',#6574,'design');
#6502=PRODUCT_DEFINITION('Front Right Z Mount','Front Right Z Mount',#6526,
#6500);
#6526=PRODUCT_DEFINITION_FORMATION('',$,#6577);
#6574=APPLICATION_CONTEXT('Managed model based 3d engineering');
#6575=PRODUCT_CONTEXT('part definition',#6574,'mechanical');
#6577=PRODUCT('Front Right Z Mount','Front Right Z Mount',
'LEGAL AND USAGE DISCLAIMER: this Data/Model is provided \X2\201C\X0\A
S IS\X2\201D\X0\ for informational and representational only. It is a 
geometric approximation and is NOT engineered, certified, or guarantee
d for dimensional accuracy, exact tolerances, or production-level prec
ision. Vendor disclaims all implied warranties including fitness for a
 particular purpose. DO NOT USE FOR DIRECT PHYSICAL MANUFACTURING, AUT
OMATED PRODUCTION, OR SAFETY-CRITICAL SYSTEMS without independent engi
neering verification and resolution of any design discrepancies.',(#6575));
#6601=PRESENTATION_STYLE_ASSIGNMENT((#6607));
#6607=SURFACE_STYLE_USAGE(.BOTH.,#6613);
#6613=SURFACE_SIDE_STYLE('',(#6619));
#6619=SURFACE_STYLE_FILL_AREA(#6625);
#6625=FILL_AREA_STYLE('Opaque(179,179,179)',(#6631));
#6631=FILL_AREA_STYLE_COLOUR('Opaque(179,179,179)',#6637);
#6637=COLOUR_RGB('Opaque(179,179,179)',0.701960784313725,0.701960784313725,
0.701960784313725);
ENDSEC;
END-ISO-10303-21;
